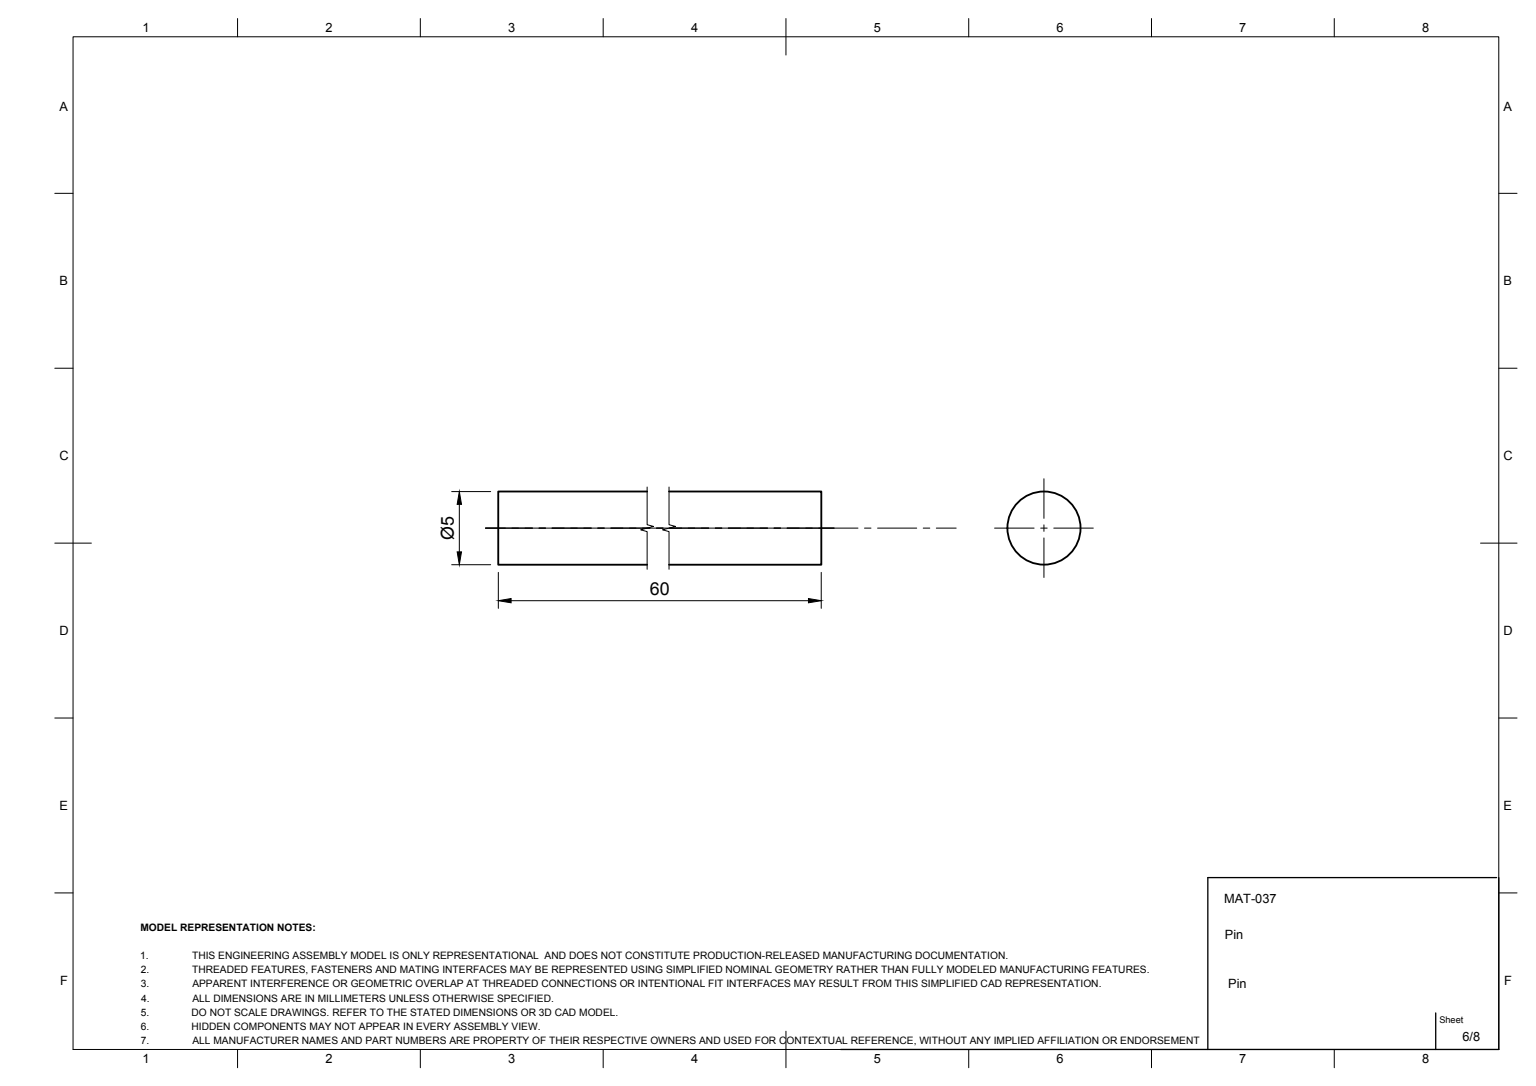
ISO-10303-21;
HEADER;
/* Generated by software containing ST-Developer
 * from STEP Tools, Inc. (www.steptools.com) 
 */

FILE_DESCRIPTION(
/* description */ ('STEP AP214'),
/* implementation_level */ '2;1');

FILE_NAME(
/* name */ 'PIN.step',
/* time_stamp */ '2026-11-14T21:09:07-08:00',
/* author */ (''),
/* organization */ (''),
/* preprocessor_version */ 'ST-DEVELOPER v20.2',
/* originating_system */ 'Autodesk Translation Framework v15.17.0.0',
/* authorisation */ '');

FILE_SCHEMA (('AUTOMOTIVE_DESIGN { 1 0 10303 214 3 1 1 }'));
ENDSEC;

DATA;
#10=MECHANICAL_DESIGN_GEOMETRIC_PRESENTATION_REPRESENTATION('',(#82),#2059);
#68=SHAPE_REPRESENTATION_RELATIONSHIP('SRR','None',#2098,#75);
#75=ADVANCED_BREP_SHAPE_REPRESENTATION('',(#89),#2056);
#82=STYLED_ITEM('',(#2142),#89);
#89=MANIFOLD_SOLID_BREP('Body1',#979);
#114=PLANE('',#1141);
#115=PLANE('',#1142);
#196=FACE_OUTER_BOUND('',#272,.T.);
#197=FACE_OUTER_BOUND('',#273,.T.);
#198=FACE_OUTER_BOUND('',#274,.T.);
#272=EDGE_LOOP('',(#837,#838,#839,#840));
#273=EDGE_LOOP('',(#841));
#274=EDGE_LOOP('',(#842));
#335=LINE('',#1952,#400);
#400=VECTOR('',#1387,2.49999999999999);
#450=CIRCLE('',#1139,2.49999999999999);
#451=CIRCLE('',#1140,2.49999999999999);
#520=VERTEX_POINT('',#1949);
#521=VERTEX_POINT('',#1951);
#629=EDGE_CURVE('',#520,#520,#450,.T.);
#630=EDGE_CURVE('',#520,#521,#335,.T.);
#631=EDGE_CURVE('',#521,#521,#451,.T.);
#837=ORIENTED_EDGE('',*,*,#629,.T.);
#838=ORIENTED_EDGE('',*,*,#630,.T.);
#839=ORIENTED_EDGE('',*,*,#631,.F.);
#840=ORIENTED_EDGE('',*,*,#630,.F.);
#841=ORIENTED_EDGE('',*,*,#631,.T.);
#842=ORIENTED_EDGE('',*,*,#629,.F.);
#914=CYLINDRICAL_SURFACE('',#1138,2.49999999999999);
#959=ADVANCED_FACE('',(#196),#914,.T.);
#960=ADVANCED_FACE('',(#197),#114,.T.);
#961=ADVANCED_FACE('',(#198),#115,.F.);
#979=CLOSED_SHELL('',(#959,#960,#961));
#1137=AXIS2_PLACEMENT_3D('',#1947,#1381,#1382);
#1138=AXIS2_PLACEMENT_3D('',#1948,#1383,#1384);
#1139=AXIS2_PLACEMENT_3D('',#1950,#1385,#1386);
#1140=AXIS2_PLACEMENT_3D('',#1953,#1388,#1389);
#1141=AXIS2_PLACEMENT_3D('',#1954,#1390,#1391);
#1142=AXIS2_PLACEMENT_3D('',#1955,#1392,#1393);
#1381=DIRECTION('axis',(0.,0.,1.));
#1382=DIRECTION('refdir',(1.,0.,0.));
#1383=DIRECTION('center_axis',(-1.06387995116713E-16,-6.73459620742395E-16,
-1.));
#1384=DIRECTION('ref_axis',(-1.,2.27595720048158E-15,1.06387995116711E-16));
#1385=DIRECTION('center_axis',(1.06387995116713E-16,6.73459620742395E-16,
1.));
#1386=DIRECTION('ref_axis',(1.,-2.27595720048158E-15,-1.06387995116711E-16));
#1387=DIRECTION('',(1.06387995116713E-16,6.73459620742395E-16,1.));
#1388=DIRECTION('center_axis',(1.06387995116713E-16,6.73459620742395E-16,
1.));
#1389=DIRECTION('ref_axis',(1.,-2.27595720048158E-15,-1.06387995116711E-16));
#1390=DIRECTION('center_axis',(-1.00785894677507E-16,6.73459620742396E-16,
1.));
#1391=DIRECTION('ref_axis',(1.,-2.27595720048158E-15,1.00785894677509E-16));
#1392=DIRECTION('center_axis',(-1.00785894677507E-16,6.73459620742396E-16,
1.));
#1393=DIRECTION('ref_axis',(1.,-2.27595720048158E-15,1.00785894677509E-16));
#1947=CARTESIAN_POINT('',(0.,0.,0.));
#1948=CARTESIAN_POINT('Origin',(0.,-5.55111512312578E-14,60.0000000000028));
#1949=CARTESIAN_POINT('',(2.49999999999999,-1.01914783176794E-13,0.));
#1950=CARTESIAN_POINT('Origin',(0.,0.,0.));
#1951=CARTESIAN_POINT('',(2.49999999999999,-6.15072059322486E-14,60.0000000000028));
#1952=CARTESIAN_POINT('',(2.49999999999999,-6.15072059322486E-14,60.0000000000028));
#1953=CARTESIAN_POINT('Origin',(0.,-5.55111512312578E-14,60.0000000000028));
#1954=CARTESIAN_POINT('Origin',(0.,-5.55111512312578E-14,60.0000000000028));
#1955=CARTESIAN_POINT('Origin',(0.,0.,0.));
#2047=UNCERTAINTY_MEASURE_WITH_UNIT(LENGTH_MEASURE(0.01),#2060,
'DISTANCE_ACCURACY_VALUE',
'Maximum model space distance between geometric entities at asserted c
onnectivities');
#2050=UNCERTAINTY_MEASURE_WITH_UNIT(LENGTH_MEASURE(0.01),#2060,
'DISTANCE_ACCURACY_VALUE',
'Maximum model space distance between geometric entities at asserted c
onnectivities');
#2056=(
GEOMETRIC_REPRESENTATION_CONTEXT(3)
GLOBAL_UNCERTAINTY_ASSIGNED_CONTEXT((#2047))
GLOBAL_UNIT_ASSIGNED_CONTEXT((#2060,#2062,#2063))
REPRESENTATION_CONTEXT('','3D')
);
#2059=(
GEOMETRIC_REPRESENTATION_CONTEXT(3)
GLOBAL_UNCERTAINTY_ASSIGNED_CONTEXT((#2050))
GLOBAL_UNIT_ASSIGNED_CONTEXT((#2060,#2062,#2063))
REPRESENTATION_CONTEXT('','3D')
);
#2060=(
LENGTH_UNIT()
NAMED_UNIT(*)
SI_UNIT(.MILLI.,.METRE.)
);
#2062=(
NAMED_UNIT(*)
PLANE_ANGLE_UNIT()
SI_UNIT($,.RADIAN.)
);
#2063=(
NAMED_UNIT(*)
SI_UNIT($,.STERADIAN.)
SOLID_ANGLE_UNIT()
);
#2069=SHAPE_DEFINITION_REPRESENTATION(#2077,#2098);
#2077=PRODUCT_DEFINITION_SHAPE('',$,#2107);
#2098=SHAPE_REPRESENTATION('',(#1137),#2056);
#2101=PRODUCT_DEFINITION_CONTEXT('part definition',#2127,'design');
#2107=PRODUCT_DEFINITION('Pin','PIN',#2115,#2101);
#2115=PRODUCT_DEFINITION_FORMATION('',$,#2134);
#2127=APPLICATION_CONTEXT(
'Core Data for Automotive Mechanical Design Process');
#2128=PRODUCT_CONTEXT('part definition',#2127,'mechanical');
#2134=PRODUCT('Pin','PIN',$,(#2128));
#2142=PRESENTATION_STYLE_ASSIGNMENT((#2148));
#2148=SURFACE_STYLE_USAGE(.BOTH.,#2154);
#2154=SURFACE_SIDE_STYLE('',(#2160));
#2160=SURFACE_STYLE_FILL_AREA(#2166);
#2166=FILL_AREA_STYLE('Opaque(122,133,145)',(#2172));
#2172=FILL_AREA_STYLE_COLOUR('Opaque(122,133,145)',#2178);
#2178=COLOUR_RGB('Opaque(122,133,145)',0.47843137254902,0.52156862745098,
0.568627450980392);
ENDSEC;
END-ISO-10303-21;
